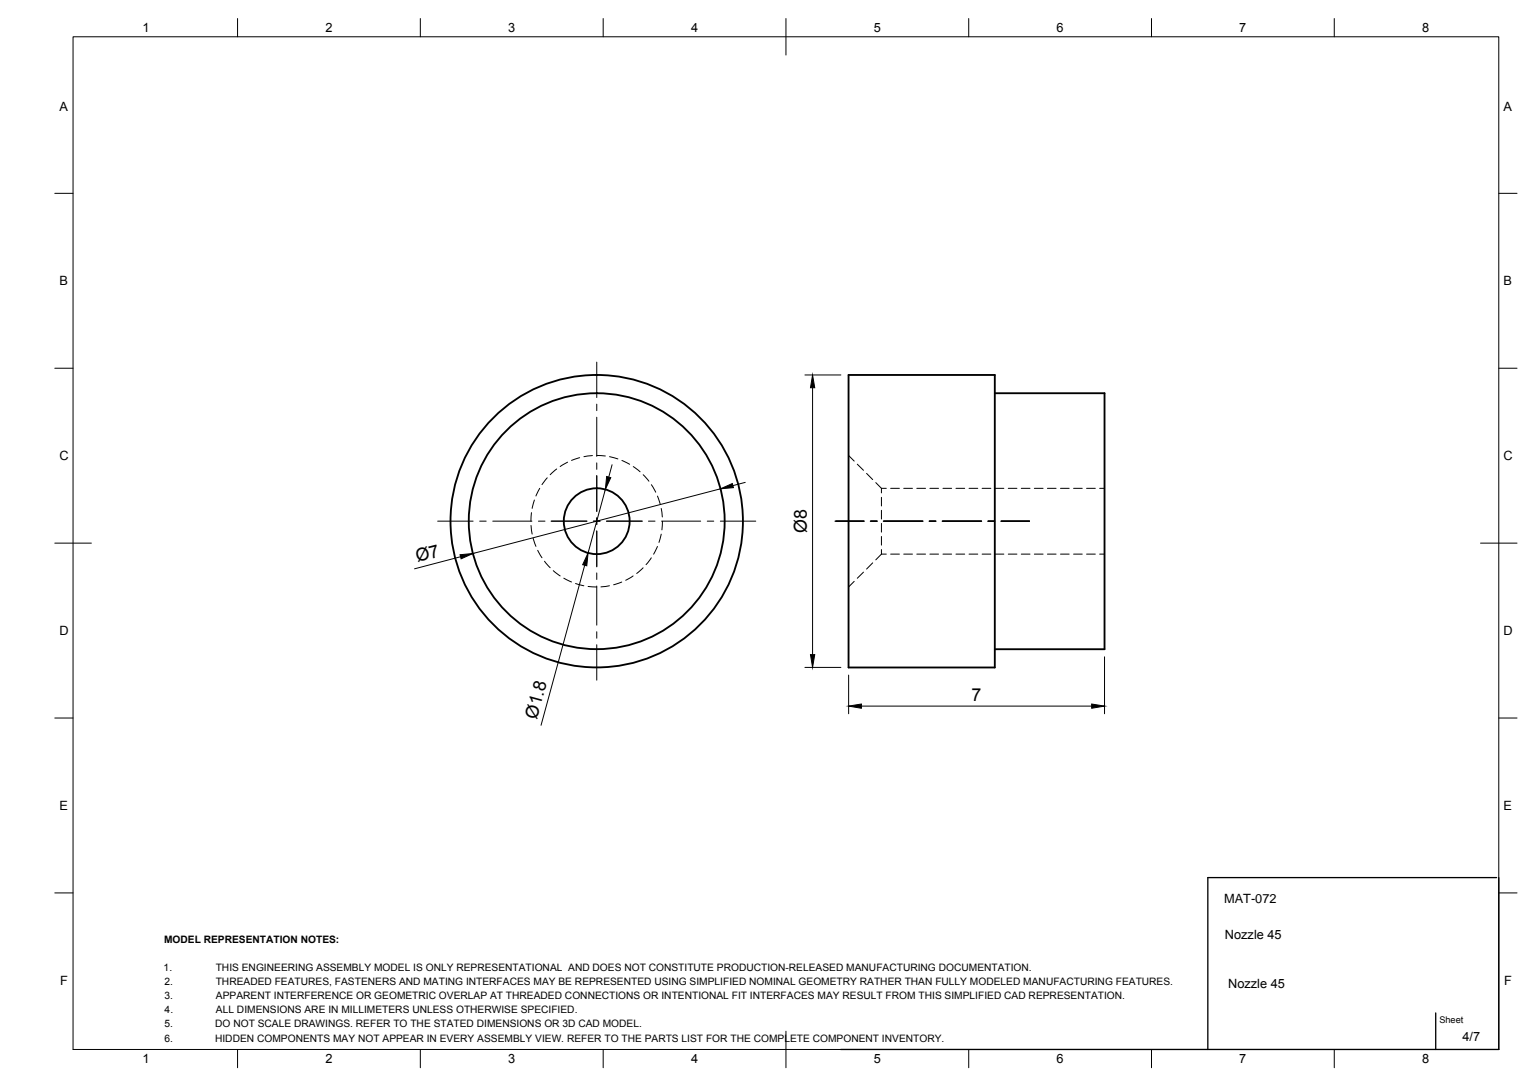
ISO-10303-21;
HEADER;
/* Generated by software containing ST-Developer
 * from STEP Tools, Inc. (www.steptools.com) 
 */

FILE_DESCRIPTION(
/* description */ (''),
/* implementation_level */ '2;1');

FILE_NAME(
/* name */ 'Nozzle 45.step',
/* time_stamp */ '2026-10-24T10:30:45-07:00',
/* author */ (''),
/* organization */ (''),
/* preprocessor_version */ 'ST-DEVELOPER v20.2',
/* originating_system */ 'Autodesk Translation Framework v15.15.0.0',
/* authorisation */ '');

FILE_SCHEMA (('AUTOMOTIVE_DESIGN { 1 0 10303 214 3 1 1 }'));
ENDSEC;

DATA;
#10=MECHANICAL_DESIGN_GEOMETRIC_PRESENTATION_REPRESENTATION('',(#78),#5183);
#63=CONICAL_SURFACE('',#2616,1.8,0.785398163397447);
#68=SHAPE_REPRESENTATION_RELATIONSHIP('SRR','None',#5215,#73);
#73=ADVANCED_BREP_SHAPE_REPRESENTATION('',(#83),#5179);
#78=STYLED_ITEM('',(#5247),#83);
#83=MANIFOLD_SOLID_BREP('Nozzle 45',#2364);
#132=FACE_BOUND('',#568,.T.);
#133=FACE_BOUND('',#570,.T.);
#134=FACE_BOUND('',#574,.T.);
#194=PLANE('',#2609);
#195=PLANE('',#2611);
#196=PLANE('',#2617);
#384=FACE_OUTER_BOUND('',#566,.T.);
#385=FACE_OUTER_BOUND('',#567,.T.);
#386=FACE_OUTER_BOUND('',#569,.T.);
#387=FACE_OUTER_BOUND('',#571,.T.);
#388=FACE_OUTER_BOUND('',#572,.T.);
#389=FACE_OUTER_BOUND('',#573,.T.);
#390=FACE_OUTER_BOUND('',#575,.T.);
#566=EDGE_LOOP('',(#2064,#2065,#2066,#2067));
#567=EDGE_LOOP('',(#2068));
#568=EDGE_LOOP('',(#2069));
#569=EDGE_LOOP('',(#2070));
#570=EDGE_LOOP('',(#2071));
#571=EDGE_LOOP('',(#2072,#2073,#2074,#2075));
#572=EDGE_LOOP('',(#2076,#2077,#2078,#2079));
#573=EDGE_LOOP('',(#2080));
#574=EDGE_LOOP('',(#2081));
#575=EDGE_LOOP('',(#2082,#2083,#2084,#2085));
#676=CIRCLE('',#2607,4.00000000000001);
#677=CIRCLE('',#2608,4.00000000000001);
#678=CIRCLE('',#2610,3.50000000000001);
#679=CIRCLE('',#2612,1.8);
#680=CIRCLE('',#2614,0.899999999999997);
#681=CIRCLE('',#2615,0.899999999999995);
#682=CIRCLE('',#2618,3.50000000000001);
#838=LINE('',#5058,#988);
#839=LINE('',#5070,#989);
#840=LINE('',#5073,#990);
#841=LINE('',#5078,#991);
#988=VECTOR('',#3180,4.00000000000001);
#989=VECTOR('',#3195,0.899999999999993);
#990=VECTOR('',#3200,1.8);
#991=VECTOR('',#3207,3.50000000000002);
#1182=VERTEX_POINT('',#5055);
#1183=VERTEX_POINT('',#5057);
#1184=VERTEX_POINT('',#5061);
#1185=VERTEX_POINT('',#5064);
#1186=VERTEX_POINT('',#5067);
#1187=VERTEX_POINT('',#5069);
#1188=VERTEX_POINT('',#5075);
#1480=EDGE_CURVE('',#1182,#1182,#676,.T.);
#1481=EDGE_CURVE('',#1182,#1183,#838,.T.);
#1482=EDGE_CURVE('',#1183,#1183,#677,.T.);
#1483=EDGE_CURVE('',#1184,#1184,#678,.T.);
#1484=EDGE_CURVE('',#1185,#1185,#679,.T.);
#1485=EDGE_CURVE('',#1186,#1186,#680,.T.);
#1486=EDGE_CURVE('',#1186,#1187,#839,.T.);
#1487=EDGE_CURVE('',#1187,#1187,#681,.T.);
#1488=EDGE_CURVE('',#1187,#1185,#840,.T.);
#1489=EDGE_CURVE('',#1188,#1188,#682,.T.);
#1490=EDGE_CURVE('',#1184,#1188,#841,.T.);
#2064=ORIENTED_EDGE('',*,*,#1480,.T.);
#2065=ORIENTED_EDGE('',*,*,#1481,.T.);
#2066=ORIENTED_EDGE('',*,*,#1482,.F.);
#2067=ORIENTED_EDGE('',*,*,#1481,.F.);
#2068=ORIENTED_EDGE('',*,*,#1482,.T.);
#2069=ORIENTED_EDGE('',*,*,#1483,.F.);
#2070=ORIENTED_EDGE('',*,*,#1480,.F.);
#2071=ORIENTED_EDGE('',*,*,#1484,.F.);
#2072=ORIENTED_EDGE('',*,*,#1485,.T.);
#2073=ORIENTED_EDGE('',*,*,#1486,.T.);
#2074=ORIENTED_EDGE('',*,*,#1487,.T.);
#2075=ORIENTED_EDGE('',*,*,#1486,.F.);
#2076=ORIENTED_EDGE('',*,*,#1487,.F.);
#2077=ORIENTED_EDGE('',*,*,#1488,.T.);
#2078=ORIENTED_EDGE('',*,*,#1484,.T.);
#2079=ORIENTED_EDGE('',*,*,#1488,.F.);
#2080=ORIENTED_EDGE('',*,*,#1489,.T.);
#2081=ORIENTED_EDGE('',*,*,#1485,.F.);
#2082=ORIENTED_EDGE('',*,*,#1483,.T.);
#2083=ORIENTED_EDGE('',*,*,#1490,.T.);
#2084=ORIENTED_EDGE('',*,*,#1489,.F.);
#2085=ORIENTED_EDGE('',*,*,#1490,.F.);
#2211=CYLINDRICAL_SURFACE('',#2606,4.00000000000001);
#2212=CYLINDRICAL_SURFACE('',#2613,0.899999999999993);
#2213=CYLINDRICAL_SURFACE('',#2619,3.50000000000001);
#2335=ADVANCED_FACE('',(#384),#2211,.T.);
#2336=ADVANCED_FACE('',(#385,#132),#194,.T.);
#2337=ADVANCED_FACE('',(#386,#133),#195,.F.);
#2338=ADVANCED_FACE('',(#387),#2212,.F.);
#2339=ADVANCED_FACE('',(#388),#63,.F.);
#2340=ADVANCED_FACE('',(#389,#134),#196,.T.);
#2341=ADVANCED_FACE('',(#390),#2213,.T.);
#2364=CLOSED_SHELL('',(#2335,#2336,#2337,#2338,#2339,#2340,#2341));
#2605=AXIS2_PLACEMENT_3D('',#5053,#3174,#3175);
#2606=AXIS2_PLACEMENT_3D('',#5054,#3176,#3177);
#2607=AXIS2_PLACEMENT_3D('',#5056,#3178,#3179);
#2608=AXIS2_PLACEMENT_3D('',#5059,#3181,#3182);
#2609=AXIS2_PLACEMENT_3D('',#5060,#3183,#3184);
#2610=AXIS2_PLACEMENT_3D('',#5062,#3185,#3186);
#2611=AXIS2_PLACEMENT_3D('',#5063,#3187,#3188);
#2612=AXIS2_PLACEMENT_3D('',#5065,#3189,#3190);
#2613=AXIS2_PLACEMENT_3D('',#5066,#3191,#3192);
#2614=AXIS2_PLACEMENT_3D('',#5068,#3193,#3194);
#2615=AXIS2_PLACEMENT_3D('',#5071,#3196,#3197);
#2616=AXIS2_PLACEMENT_3D('',#5072,#3198,#3199);
#2617=AXIS2_PLACEMENT_3D('',#5074,#3201,#3202);
#2618=AXIS2_PLACEMENT_3D('',#5076,#3203,#3204);
#2619=AXIS2_PLACEMENT_3D('',#5077,#3205,#3206);
#3174=DIRECTION('axis',(0.,0.,1.));
#3175=DIRECTION('refdir',(1.,0.,0.));
#3176=DIRECTION('center_axis',(-0.612372435695796,0.707106781186546,-0.353553390593275));
#3177=DIRECTION('ref_axis',(-0.755928946018453,-0.654653670707979,0.));
#3178=DIRECTION('center_axis',(0.612372435695796,-0.707106781186546,0.353553390593275));
#3179=DIRECTION('ref_axis',(0.755928946018453,0.654653670707979,0.));
#3180=DIRECTION('',(0.612372435695796,-0.707106781186546,0.353553390593275));
#3181=DIRECTION('center_axis',(0.612372435695796,-0.707106781186546,0.353553390593275));
#3182=DIRECTION('ref_axis',(0.755928946018453,0.654653670707979,0.));
#3183=DIRECTION('center_axis',(0.612372435695796,-0.707106781186546,0.353553390593275));
#3184=DIRECTION('ref_axis',(0.5,0.,-0.866025403784438));
#3185=DIRECTION('center_axis',(0.612372435695796,-0.707106781186546,0.353553390593275));
#3186=DIRECTION('ref_axis',(0.755928946018453,0.654653670707979,0.));
#3187=DIRECTION('center_axis',(0.612372435695796,-0.707106781186546,0.353553390593275));
#3188=DIRECTION('ref_axis',(0.5,0.,-0.866025403784438));
#3189=DIRECTION('center_axis',(-0.612372435695796,0.707106781186546,-0.353553390593275));
#3190=DIRECTION('ref_axis',(-0.755928946018453,-0.654653670707979,0.));
#3191=DIRECTION('center_axis',(-0.612372435695796,0.707106781186546,-0.353553390593275));
#3192=DIRECTION('ref_axis',(-0.755928946018453,-0.654653670707979,0.));
#3193=DIRECTION('center_axis',(0.612372435695796,-0.707106781186546,0.353553390593275));
#3194=DIRECTION('ref_axis',(0.755928946018453,0.654653670707979,0.));
#3195=DIRECTION('',(-0.612372435695796,0.707106781186546,-0.353553390593275));
#3196=DIRECTION('center_axis',(-0.612372435695796,0.707106781186546,-0.353553390593275));
#3197=DIRECTION('ref_axis',(-0.755928946018453,-0.654653670707979,0.));
#3198=DIRECTION('center_axis',(-0.612372435695796,0.707106781186546,-0.353553390593275));
#3199=DIRECTION('ref_axis',(-0.755928946018453,-0.654653670707979,0.));
#3200=DIRECTION('',(0.101509781932626,0.962910049886276,-0.250000000000001));
#3201=DIRECTION('center_axis',(0.612372435695796,-0.707106781186546,0.353553390593275));
#3202=DIRECTION('ref_axis',(0.5,0.,-0.866025403784438));
#3203=DIRECTION('center_axis',(0.612372435695796,-0.707106781186546,0.353553390593275));
#3204=DIRECTION('ref_axis',(0.755928946018453,0.654653670707979,0.));
#3205=DIRECTION('center_axis',(-0.612372435695796,0.707106781186546,-0.353553390593275));
#3206=DIRECTION('ref_axis',(-0.755928946018453,-0.654653670707979,0.));
#3207=DIRECTION('',(0.612372435695796,-0.707106781186546,0.353553390593275));
#5053=CARTESIAN_POINT('',(0.,0.,0.));
#5054=CARTESIAN_POINT('Origin',(-116.12807069331,130.343145750508,-79.0465728752519));
#5055=CARTESIAN_POINT('',(-115.553844652019,135.790187558086,-80.460786437625));
#5056=CARTESIAN_POINT('Origin',(-118.577560436093,133.171572875254,-80.460786437625));
#5057=CARTESIAN_POINT('',(-113.104354909236,132.96176043334,-79.0465728752519));
#5058=CARTESIAN_POINT('',(-113.104354909236,132.96176043334,-79.0465728752519));
#5059=CARTESIAN_POINT('Origin',(-116.12807069331,130.343145750508,-79.0465728752519));
#5060=CARTESIAN_POINT('Origin',(-116.12807069331,130.343145750508,-79.0465728752519));
#5061=CARTESIAN_POINT('',(-113.482319382245,132.634433597986,-79.0465728752519));
#5062=CARTESIAN_POINT('Origin',(-116.12807069331,130.343145750508,-79.0465728752519));
#5063=CARTESIAN_POINT('Origin',(-118.577560436093,133.171572875254,-80.460786437625));
#5064=CARTESIAN_POINT('',(-117.21688833326,134.349949482528,-80.460786437625));
#5065=CARTESIAN_POINT('Origin',(-118.577560436093,133.171572875254,-80.460786437625));
#5066=CARTESIAN_POINT('Origin',(-118.577560436093,133.171572875254,-80.460786437625));
#5067=CARTESIAN_POINT('',(-113.610617334806,128.811013710585,-77.9859127034721));
#5068=CARTESIAN_POINT('Origin',(-114.290953386223,128.221825406948,-77.9859127034721));
#5069=CARTESIAN_POINT('',(-117.34608919255,133.124365075823,-80.1425883860911));
#5070=CARTESIAN_POINT('',(-117.897224384677,133.760761178891,-80.460786437625));
#5071=CARTESIAN_POINT('Origin',(-118.026425243967,132.535176772186,-80.1425883860911));
#5072=CARTESIAN_POINT('Origin',(-118.577560436093,133.171572875254,-80.460786437625));
#5073=CARTESIAN_POINT('',(-117.21688833326,134.349949482528,-80.460786437625));
#5074=CARTESIAN_POINT('Origin',(-114.290953386223,128.221825406948,-77.9859127034721));
#5075=CARTESIAN_POINT('',(-111.645202075158,130.513113254426,-77.9859127034721));
#5076=CARTESIAN_POINT('Origin',(-114.290953386223,128.221825406948,-77.9859127034721));
#5077=CARTESIAN_POINT('Origin',(-114.290953386223,128.221825406948,-77.9859127034721));
#5078=CARTESIAN_POINT('',(-111.645202075158,130.513113254426,-77.9859127034721));
#5172=UNCERTAINTY_MEASURE_WITH_UNIT(LENGTH_MEASURE(0.01),#5184,
'DISTANCE_ACCURACY_VALUE',
'Maximum model space distance between geometric entities at asserted c
onnectivities');
#5176=UNCERTAINTY_MEASURE_WITH_UNIT(LENGTH_MEASURE(0.01),#5184,
'DISTANCE_ACCURACY_VALUE',
'Maximum model space distance between geometric entities at asserted c
onnectivities');
#5179=(
GEOMETRIC_REPRESENTATION_CONTEXT(3)
GLOBAL_UNCERTAINTY_ASSIGNED_CONTEXT((#5172))
GLOBAL_UNIT_ASSIGNED_CONTEXT((#5184,#5186,#5187))
REPRESENTATION_CONTEXT('','3D')
);
#5183=(
GEOMETRIC_REPRESENTATION_CONTEXT(3)
GLOBAL_UNCERTAINTY_ASSIGNED_CONTEXT((#5176))
GLOBAL_UNIT_ASSIGNED_CONTEXT((#5184,#5186,#5187))
REPRESENTATION_CONTEXT('','3D')
);
#5184=(
LENGTH_UNIT()
NAMED_UNIT(*)
SI_UNIT(.MILLI.,.METRE.)
);
#5186=(
NAMED_UNIT(*)
PLANE_ANGLE_UNIT()
SI_UNIT($,.RADIAN.)
);
#5187=(
NAMED_UNIT(*)
SI_UNIT($,.STERADIAN.)
SOLID_ANGLE_UNIT()
);
#5190=SHAPE_DEFINITION_REPRESENTATION(#5196,#5215);
#5196=PRODUCT_DEFINITION_SHAPE('',$,#5222);
#5215=SHAPE_REPRESENTATION('',(#2605),#5179);
#5219=PRODUCT_DEFINITION_CONTEXT('part definition',#5239,'design');
#5222=PRODUCT_DEFINITION('Nozzle 45','Nozzle 45',#5228,#5219);
#5228=PRODUCT_DEFINITION_FORMATION('',$,#5243);
#5239=APPLICATION_CONTEXT(
'Core Data for Automotive Mechanical Design Process');
#5240=PRODUCT_CONTEXT('part definition',#5239,'mechanical');
#5243=PRODUCT('Nozzle 45','Nozzle 45',$,(#5240));
#5247=PRESENTATION_STYLE_ASSIGNMENT((#5248));
#5248=SURFACE_STYLE_USAGE(.BOTH.,#5249);
#5249=SURFACE_SIDE_STYLE('',(#5250));
#5250=SURFACE_STYLE_FILL_AREA(#5251);
#5251=FILL_AREA_STYLE('Steel - Satin',(#5252));
#5252=FILL_AREA_STYLE_COLOUR('Steel - Satin',#5253);
#5253=COLOUR_RGB('Steel - Satin',0.627450980392157,0.627450980392157,0.627450980392157);
ENDSEC;
END-ISO-10303-21;
